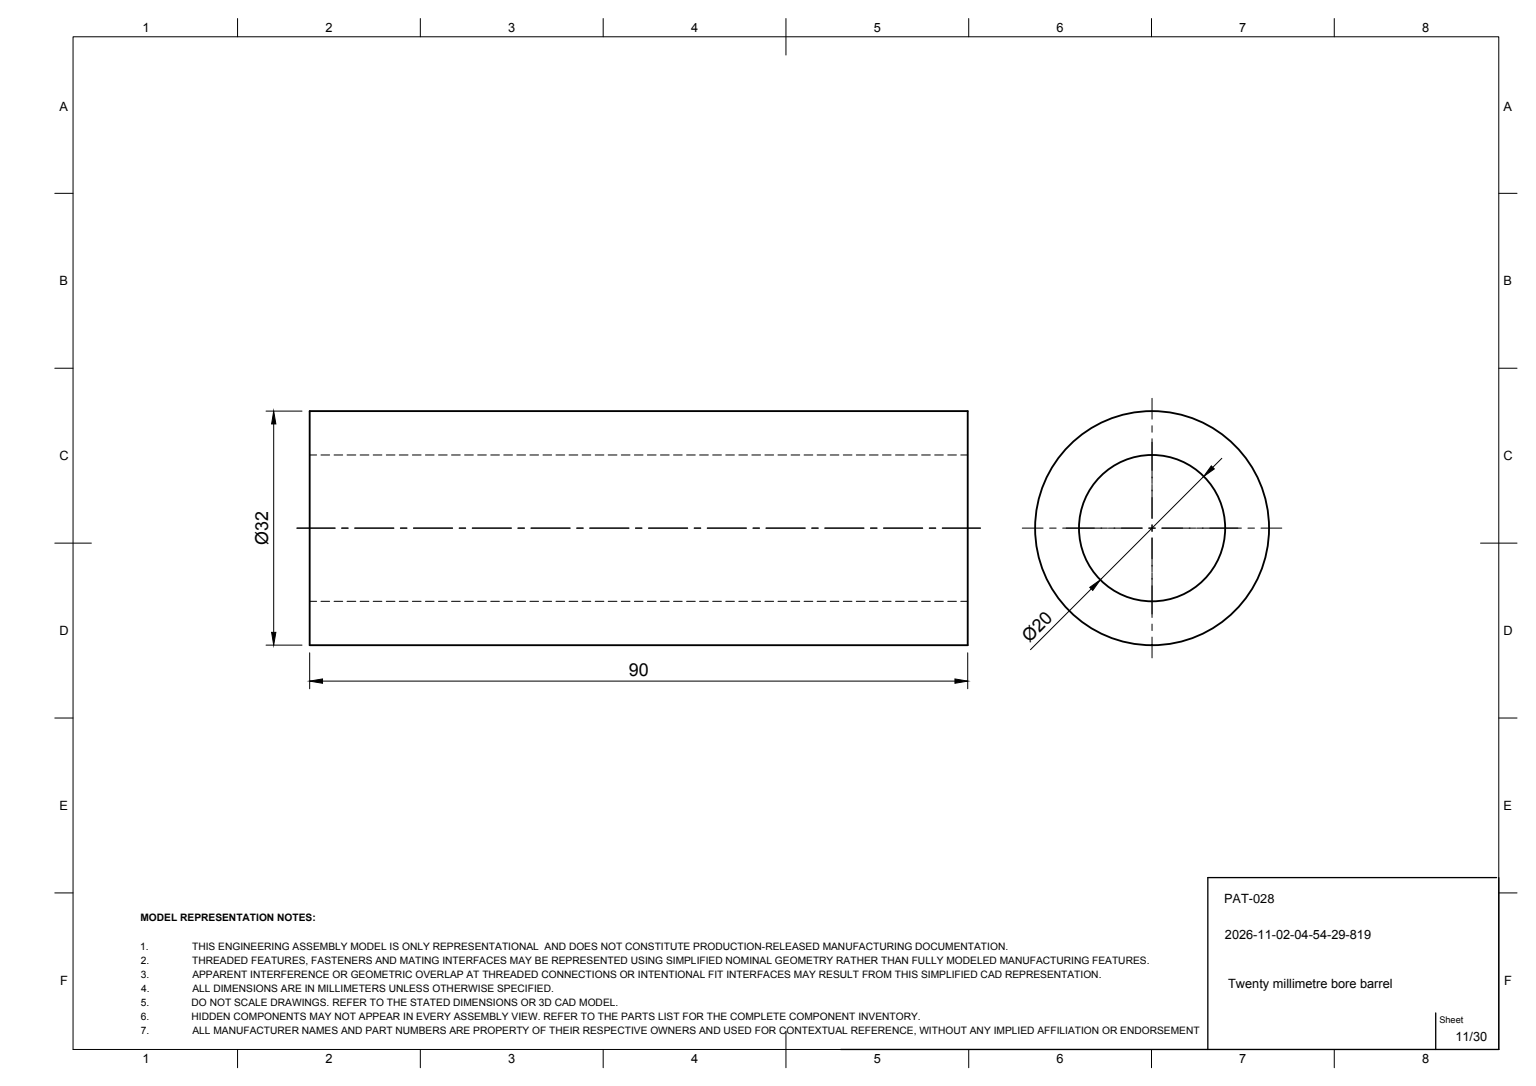
ISO-10303-21;
HEADER;
/* Generated by software containing ST-Developer
 * from STEP Tools, Inc. (www.steptools.com) 
 */

FILE_DESCRIPTION(
/* description */ ('Cylinder foot and clevis mount kit'),
/* implementation_level */ '2;1');

FILE_NAME(
/* name */ 'Twenty millimetre bore barrel.step',
/* time_stamp */ '2026-10-27T20:10:43-07:00',
/* author */ (''),
/* organization */ (''),
/* preprocessor_version */ 'ST-DEVELOPER v20.2',
/* originating_system */ 'Autodesk Translation Framework v15.17.0.0',
/* authorisation */ '');

FILE_SCHEMA (('AUTOMOTIVE_DESIGN { 1 0 10303 214 3 1 1 }'));
ENDSEC;

DATA;
#10=MECHANICAL_DESIGN_GEOMETRIC_PRESENTATION_REPRESENTATION('',(#344),#9102);
#288=SHAPE_REPRESENTATION_RELATIONSHIP('SRR','None',#9235,#316);
#316=ADVANCED_BREP_SHAPE_REPRESENTATION('',(#372),#9078);
#344=STYLED_ITEM('',(#9453),#372);
#372=MANIFOLD_SOLID_BREP('Body1',#4930);
#440=FACE_BOUND('',#1185,.T.);
#441=FACE_BOUND('',#1187,.T.);
#591=PLANE('',#5521);
#592=PLANE('',#5522);
#828=FACE_OUTER_BOUND('',#1182,.T.);
#829=FACE_OUTER_BOUND('',#1183,.T.);
#830=FACE_OUTER_BOUND('',#1184,.T.);
#831=FACE_OUTER_BOUND('',#1186,.T.);
#1182=EDGE_LOOP('',(#3861,#3862,#3863,#3864));
#1183=EDGE_LOOP('',(#3865,#3866,#3867,#3868));
#1184=EDGE_LOOP('',(#3869));
#1185=EDGE_LOOP('',(#3870));
#1186=EDGE_LOOP('',(#3871));
#1187=EDGE_LOOP('',(#3872));
#1573=LINE('',#8085,#1922);
#1574=LINE('',#8091,#1923);
#1922=VECTOR('',#6562,1.);
#1923=VECTOR('',#6569,1.6);
#2204=CIRCLE('',#5516,1.);
#2205=CIRCLE('',#5517,1.);
#2206=CIRCLE('',#5519,1.6);
#2207=CIRCLE('',#5520,1.6);
#2498=VERTEX_POINT('',#8082);
#2499=VERTEX_POINT('',#8084);
#2500=VERTEX_POINT('',#8088);
#2501=VERTEX_POINT('',#8090);
#2985=EDGE_CURVE('',#2498,#2498,#2204,.T.);
#2986=EDGE_CURVE('',#2498,#2499,#1573,.T.);
#2987=EDGE_CURVE('',#2499,#2499,#2205,.T.);
#2988=EDGE_CURVE('',#2500,#2500,#2206,.T.);
#2989=EDGE_CURVE('',#2500,#2501,#1574,.T.);
#2990=EDGE_CURVE('',#2501,#2501,#2207,.T.);
#3861=ORIENTED_EDGE('',*,*,#2985,.F.);
#3862=ORIENTED_EDGE('',*,*,#2986,.T.);
#3863=ORIENTED_EDGE('',*,*,#2987,.T.);
#3864=ORIENTED_EDGE('',*,*,#2986,.F.);
#3865=ORIENTED_EDGE('',*,*,#2988,.F.);
#3866=ORIENTED_EDGE('',*,*,#2989,.T.);
#3867=ORIENTED_EDGE('',*,*,#2990,.T.);
#3868=ORIENTED_EDGE('',*,*,#2989,.F.);
#3869=ORIENTED_EDGE('',*,*,#2988,.T.);
#3870=ORIENTED_EDGE('',*,*,#2985,.T.);
#3871=ORIENTED_EDGE('',*,*,#2990,.F.);
#3872=ORIENTED_EDGE('',*,*,#2987,.F.);
#4568=CYLINDRICAL_SURFACE('',#5515,1.);
#4569=CYLINDRICAL_SURFACE('',#5518,1.6);
#4751=ADVANCED_FACE('',(#828),#4568,.F.);
#4752=ADVANCED_FACE('',(#829),#4569,.T.);
#4753=ADVANCED_FACE('',(#830,#440),#591,.T.);
#4754=ADVANCED_FACE('',(#831,#441),#592,.F.);
#4930=CLOSED_SHELL('',(#4751,#4752,#4753,#4754));
#5514=AXIS2_PLACEMENT_3D('',#8080,#6556,#6557);
#5515=AXIS2_PLACEMENT_3D('',#8081,#6558,#6559);
#5516=AXIS2_PLACEMENT_3D('',#8083,#6560,#6561);
#5517=AXIS2_PLACEMENT_3D('',#8086,#6563,#6564);
#5518=AXIS2_PLACEMENT_3D('',#8087,#6565,#6566);
#5519=AXIS2_PLACEMENT_3D('',#8089,#6567,#6568);
#5520=AXIS2_PLACEMENT_3D('',#8092,#6570,#6571);
#5521=AXIS2_PLACEMENT_3D('',#8093,#6572,#6573);
#5522=AXIS2_PLACEMENT_3D('',#8094,#6574,#6575);
#6556=DIRECTION('axis',(0.,0.,1.));
#6557=DIRECTION('refdir',(1.,0.,0.));
#6558=DIRECTION('center_axis',(0.,1.,0.));
#6559=DIRECTION('ref_axis',(1.,0.,0.));
#6560=DIRECTION('center_axis',(0.,-1.,0.));
#6561=DIRECTION('ref_axis',(1.,0.,0.));
#6562=DIRECTION('',(0.,-1.,0.));
#6563=DIRECTION('center_axis',(0.,-1.,0.));
#6564=DIRECTION('ref_axis',(1.,0.,0.));
#6565=DIRECTION('center_axis',(0.,1.,0.));
#6566=DIRECTION('ref_axis',(1.,0.,0.));
#6567=DIRECTION('center_axis',(0.,1.,0.));
#6568=DIRECTION('ref_axis',(1.,0.,0.));
#6569=DIRECTION('',(0.,-1.,0.));
#6570=DIRECTION('center_axis',(0.,1.,0.));
#6571=DIRECTION('ref_axis',(1.,0.,0.));
#6572=DIRECTION('center_axis',(0.,1.,0.));
#6573=DIRECTION('ref_axis',(1.,0.,0.));
#6574=DIRECTION('center_axis',(0.,1.,0.));
#6575=DIRECTION('ref_axis',(1.,0.,0.));
#8080=CARTESIAN_POINT('',(0.,0.,0.));
#8081=CARTESIAN_POINT('Origin',(0.,1.8,4.5));
#8082=CARTESIAN_POINT('',(-1.,10.8,4.5));
#8083=CARTESIAN_POINT('Origin',(0.,10.8,4.5));
#8084=CARTESIAN_POINT('',(-1.,1.8,4.5));
#8085=CARTESIAN_POINT('',(-1.,1.8,4.5));
#8086=CARTESIAN_POINT('Origin',(0.,1.8,4.5));
#8087=CARTESIAN_POINT('Origin',(0.,1.8,4.5));
#8088=CARTESIAN_POINT('',(-1.6,10.8,4.5));
#8089=CARTESIAN_POINT('Origin',(0.,10.8,4.5));
#8090=CARTESIAN_POINT('',(-1.6,1.8,4.5));
#8091=CARTESIAN_POINT('',(-1.6,1.8,4.5));
#8092=CARTESIAN_POINT('Origin',(0.,1.8,4.5));
#8093=CARTESIAN_POINT('Origin',(0.,10.8,4.5));
#8094=CARTESIAN_POINT('Origin',(0.,1.8,4.5));
#9045=UNCERTAINTY_MEASURE_WITH_UNIT(LENGTH_MEASURE(0.001),#9103,
'DISTANCE_ACCURACY_VALUE',
'Maximum model space distance between geometric entities at asserted c
onnectivities');
#9069=UNCERTAINTY_MEASURE_WITH_UNIT(LENGTH_MEASURE(0.001),#9103,
'DISTANCE_ACCURACY_VALUE',
'Maximum model space distance between geometric entities at asserted c
onnectivities');
#9078=(
GEOMETRIC_REPRESENTATION_CONTEXT(3)
GLOBAL_UNCERTAINTY_ASSIGNED_CONTEXT((#9045))
GLOBAL_UNIT_ASSIGNED_CONTEXT((#9103,#9105,#9106))
REPRESENTATION_CONTEXT('','3D')
);
#9102=(
GEOMETRIC_REPRESENTATION_CONTEXT(3)
GLOBAL_UNCERTAINTY_ASSIGNED_CONTEXT((#9069))
GLOBAL_UNIT_ASSIGNED_CONTEXT((#9103,#9105,#9106))
REPRESENTATION_CONTEXT('','3D')
);
#9103=(
LENGTH_UNIT()
NAMED_UNIT(*)
SI_UNIT(.CENTI.,.METRE.)
);
#9105=(
NAMED_UNIT(*)
PLANE_ANGLE_UNIT()
SI_UNIT($,.RADIAN.)
);
#9106=(
NAMED_UNIT(*)
SI_UNIT($,.STERADIAN.)
SOLID_ANGLE_UNIT()
);
#9115=SHAPE_DEFINITION_REPRESENTATION(#9147,#9235);
#9147=PRODUCT_DEFINITION_SHAPE('',$,#9268);
#9235=SHAPE_REPRESENTATION('',(#5514),#9078);
#9259=PRODUCT_DEFINITION_CONTEXT('part definition',#9357,'design');
#9268=PRODUCT_DEFINITION('Twenty millimetre bore barrel',
'Twenty millimetre bore barrel',#9300,#9259);
#9300=PRODUCT_DEFINITION_FORMATION('',$,#9367);
#9357=APPLICATION_CONTEXT(
'Core Data for Automotive Mechanical Design Process');
#9358=PRODUCT_CONTEXT('part definition',#9357,'mechanical');
#9367=PRODUCT('Twenty millimetre bore barrel',
'Twenty millimetre bore barrel','Twenty millimetre bore barrel',(#9358));
#9447=COLOUR_RGB('Sky Blue',0.24,0.69,0.87);
#9448=FILL_AREA_STYLE_COLOUR('',#9447);
#9449=FILL_AREA_STYLE('',(#9448));
#9450=SURFACE_STYLE_FILL_AREA(#9449);
#9451=SURFACE_SIDE_STYLE('',(#9450));
#9452=SURFACE_STYLE_USAGE(.BOTH.,#9451);
#9453=PRESENTATION_STYLE_ASSIGNMENT((#9452));
ENDSEC;
END-ISO-10303-21;
